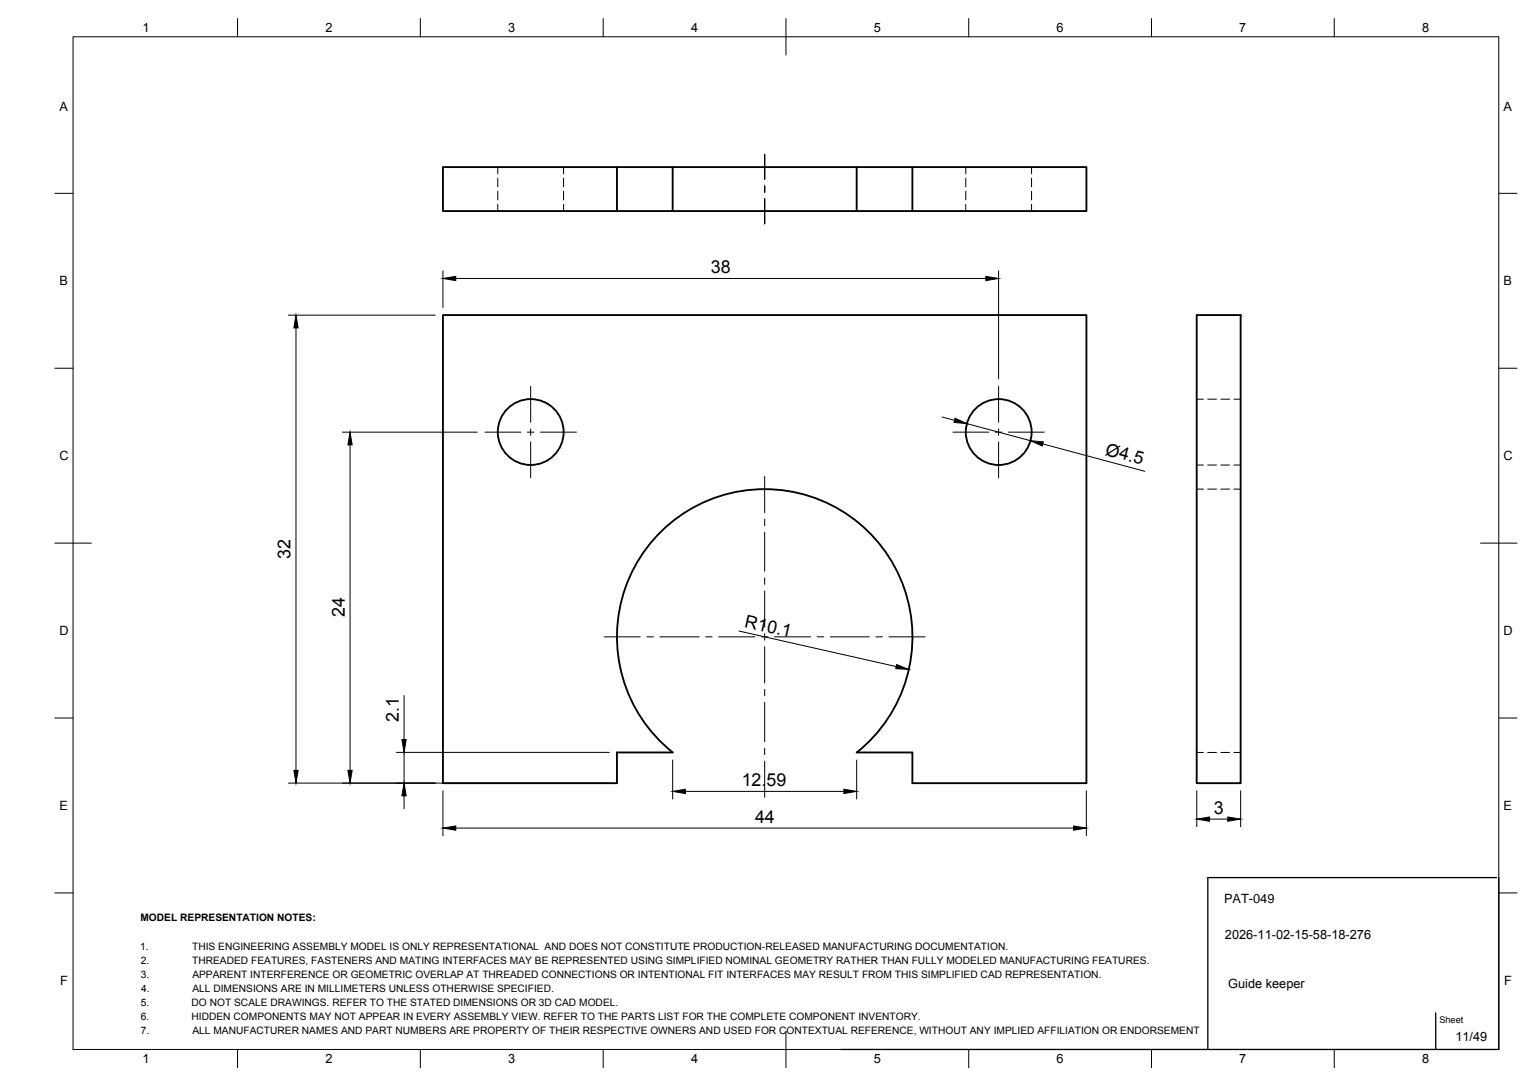
ISO-10303-21;
HEADER;
/* Generated by software containing ST-Developer
 * from STEP Tools, Inc. (www.steptools.com) 
 */

FILE_DESCRIPTION(
/* description */ ('Hand drill press frame (manual)'),
/* implementation_level */ '2;1');

FILE_NAME(
/* name */ 'Guide keeper.step',
/* time_stamp */ '2026-10-28T03:25:28-07:00',
/* author */ (''),
/* organization */ (''),
/* preprocessor_version */ 'ST-DEVELOPER v20.2',
/* originating_system */ 'Autodesk Translation Framework v15.17.0.0',
/* authorisation */ '');

FILE_SCHEMA (('AUTOMOTIVE_DESIGN { 1 0 10303 214 3 1 1 }'));
ENDSEC;

DATA;
#10=MECHANICAL_DESIGN_GEOMETRIC_PRESENTATION_REPRESENTATION('',(#625),#33299);
#535=SHAPE_REPRESENTATION_RELATIONSHIP('SRR','None',#33494,#580);
#580=ADVANCED_BREP_SHAPE_REPRESENTATION('',(#677),#33256);
#625=STYLED_ITEM('',(#33807),#677);
#677=MANIFOLD_SOLID_BREP('Body1',#12643);
#749=FACE_BOUND('',#2154,.T.);
#750=FACE_BOUND('',#2155,.T.);
#751=FACE_BOUND('',#2161,.T.);
#752=FACE_BOUND('',#2162,.T.);
#945=PLANE('',#13357);
#946=PLANE('',#13358);
#947=PLANE('',#13359);
#948=PLANE('',#13360);
#949=PLANE('',#13361);
#950=PLANE('',#13362);
#951=PLANE('',#13363);
#952=PLANE('',#13367);
#953=PLANE('',#13368);
#954=PLANE('',#13369);
#955=PLANE('',#13370);
#1427=FACE_OUTER_BOUND('',#2145,.T.);
#1428=FACE_OUTER_BOUND('',#2146,.T.);
#1429=FACE_OUTER_BOUND('',#2147,.T.);
#1430=FACE_OUTER_BOUND('',#2148,.T.);
#1431=FACE_OUTER_BOUND('',#2149,.T.);
#1432=FACE_OUTER_BOUND('',#2150,.T.);
#1433=FACE_OUTER_BOUND('',#2151,.T.);
#1434=FACE_OUTER_BOUND('',#2152,.T.);
#1435=FACE_OUTER_BOUND('',#2153,.T.);
#1436=FACE_OUTER_BOUND('',#2156,.T.);
#1437=FACE_OUTER_BOUND('',#2157,.T.);
#1438=FACE_OUTER_BOUND('',#2158,.T.);
#1439=FACE_OUTER_BOUND('',#2159,.T.);
#1440=FACE_OUTER_BOUND('',#2160,.T.);
#2145=EDGE_LOOP('',(#8835,#8836,#8837,#8838));
#2146=EDGE_LOOP('',(#8839,#8840,#8841,#8842));
#2147=EDGE_LOOP('',(#8843,#8844,#8845,#8846));
#2148=EDGE_LOOP('',(#8847,#8848,#8849,#8850));
#2149=EDGE_LOOP('',(#8851,#8852,#8853,#8854));
#2150=EDGE_LOOP('',(#8855,#8856,#8857,#8858));
#2151=EDGE_LOOP('',(#8859,#8860,#8861,#8862));
#2152=EDGE_LOOP('',(#8863,#8864,#8865,#8866));
#2153=EDGE_LOOP('',(#8867,#8868,#8869,#8870,#8871,#8872,#8873,#8874,#8875,
#8876));
#2154=EDGE_LOOP('',(#8877));
#2155=EDGE_LOOP('',(#8878));
#2156=EDGE_LOOP('',(#8879,#8880,#8881,#8882));
#2157=EDGE_LOOP('',(#8883,#8884,#8885,#8886));
#2158=EDGE_LOOP('',(#8887,#8888,#8889,#8890));
#2159=EDGE_LOOP('',(#8891,#8892,#8893,#8894));
#2160=EDGE_LOOP('',(#8895,#8896,#8897,#8898,#8899,#8900,#8901,#8902,#8903,
#8904));
#2161=EDGE_LOOP('',(#8905));
#2162=EDGE_LOOP('',(#8906));
#3015=LINE('',#18458,#4180);
#3016=LINE('',#18464,#4181);
#3017=LINE('',#18469,#4182);
#3018=LINE('',#18471,#4183);
#3019=LINE('',#18473,#4184);
#3020=LINE('',#18474,#4185);
#3021=LINE('',#18478,#4186);
#3022=LINE('',#18480,#4187);
#3023=LINE('',#18482,#4188);
#3024=LINE('',#18483,#4189);
#3025=LINE('',#18486,#4190);
#3026=LINE('',#18488,#4191);
#3027=LINE('',#18489,#4192);
#3028=LINE('',#18492,#4193);
#3029=LINE('',#18494,#4194);
#3030=LINE('',#18495,#4195);
#3031=LINE('',#18498,#4196);
#3032=LINE('',#18500,#4197);
#3033=LINE('',#18501,#4198);
#3034=LINE('',#18504,#4199);
#3035=LINE('',#18506,#4200);
#3036=LINE('',#18507,#4201);
#3037=LINE('',#18511,#4202);
#3038=LINE('',#18513,#4203);
#3039=LINE('',#18514,#4204);
#3040=LINE('',#18519,#4205);
#3041=LINE('',#18520,#4206);
#3042=LINE('',#18523,#4207);
#3043=LINE('',#18524,#4208);
#3044=LINE('',#18526,#4209);
#4180=VECTOR('',#14828,0.225);
#4181=VECTOR('',#14835,0.225);
#4182=VECTOR('',#14840,1.);
#4183=VECTOR('',#14841,1.);
#4184=VECTOR('',#14842,1.);
#4185=VECTOR('',#14843,1.);
#4186=VECTOR('',#14846,1.);
#4187=VECTOR('',#14847,1.);
#4188=VECTOR('',#14848,1.);
#4189=VECTOR('',#14849,1.);
#4190=VECTOR('',#14852,1.);
#4191=VECTOR('',#14853,1.);
#4192=VECTOR('',#14854,1.);
#4193=VECTOR('',#14857,1.);
#4194=VECTOR('',#14858,1.);
#4195=VECTOR('',#14859,1.);
#4196=VECTOR('',#14862,1.);
#4197=VECTOR('',#14863,1.);
#4198=VECTOR('',#14864,1.);
#4199=VECTOR('',#14867,1.);
#4200=VECTOR('',#14868,1.);
#4201=VECTOR('',#14869,1.);
#4202=VECTOR('',#14874,1.);
#4203=VECTOR('',#14875,1.);
#4204=VECTOR('',#14876,1.);
#4205=VECTOR('',#14883,1.);
#4206=VECTOR('',#14884,1.);
#4207=VECTOR('',#14887,1.);
#4208=VECTOR('',#14888,1.);
#4209=VECTOR('',#14891,1.);
#5280=CIRCLE('',#13352,0.225);
#5281=CIRCLE('',#13353,0.225);
#5282=CIRCLE('',#13355,0.225);
#5283=CIRCLE('',#13356,0.225);
#5284=CIRCLE('',#13364,1.01);
#5285=CIRCLE('',#13366,1.01);
#5751=VERTEX_POINT('',#18455);
#5752=VERTEX_POINT('',#18457);
#5753=VERTEX_POINT('',#18461);
#5754=VERTEX_POINT('',#18463);
#5755=VERTEX_POINT('',#18467);
#5756=VERTEX_POINT('',#18468);
#5757=VERTEX_POINT('',#18470);
#5758=VERTEX_POINT('',#18472);
#5759=VERTEX_POINT('',#18476);
#5760=VERTEX_POINT('',#18477);
#5761=VERTEX_POINT('',#18479);
#5762=VERTEX_POINT('',#18481);
#5763=VERTEX_POINT('',#18485);
#5764=VERTEX_POINT('',#18487);
#5765=VERTEX_POINT('',#18491);
#5766=VERTEX_POINT('',#18493);
#5767=VERTEX_POINT('',#18497);
#5768=VERTEX_POINT('',#18499);
#5769=VERTEX_POINT('',#18503);
#5770=VERTEX_POINT('',#18505);
#5771=VERTEX_POINT('',#18510);
#5772=VERTEX_POINT('',#18512);
#5773=VERTEX_POINT('',#18518);
#5774=VERTEX_POINT('',#18522);
#6946=EDGE_CURVE('',#5751,#5751,#5280,.T.);
#6947=EDGE_CURVE('',#5751,#5752,#3015,.T.);
#6948=EDGE_CURVE('',#5752,#5752,#5281,.T.);
#6949=EDGE_CURVE('',#5753,#5753,#5282,.T.);
#6950=EDGE_CURVE('',#5753,#5754,#3016,.T.);
#6951=EDGE_CURVE('',#5754,#5754,#5283,.T.);
#6952=EDGE_CURVE('',#5755,#5756,#3017,.T.);
#6953=EDGE_CURVE('',#5755,#5757,#3018,.T.);
#6954=EDGE_CURVE('',#5758,#5757,#3019,.T.);
#6955=EDGE_CURVE('',#5756,#5758,#3020,.T.);
#6956=EDGE_CURVE('',#5759,#5760,#3021,.T.);
#6957=EDGE_CURVE('',#5761,#5759,#3022,.T.);
#6958=EDGE_CURVE('',#5762,#5761,#3023,.T.);
#6959=EDGE_CURVE('',#5760,#5762,#3024,.T.);
#6960=EDGE_CURVE('',#5763,#5759,#3025,.T.);
#6961=EDGE_CURVE('',#5764,#5763,#3026,.T.);
#6962=EDGE_CURVE('',#5761,#5764,#3027,.T.);
#6963=EDGE_CURVE('',#5765,#5755,#3028,.T.);
#6964=EDGE_CURVE('',#5766,#5765,#3029,.T.);
#6965=EDGE_CURVE('',#5757,#5766,#3030,.T.);
#6966=EDGE_CURVE('',#5767,#5758,#3031,.T.);
#6967=EDGE_CURVE('',#5768,#5767,#3032,.T.);
#6968=EDGE_CURVE('',#5768,#5756,#3033,.T.);
#6969=EDGE_CURVE('',#5762,#5769,#3034,.T.);
#6970=EDGE_CURVE('',#5769,#5770,#3035,.T.);
#6971=EDGE_CURVE('',#5760,#5770,#3036,.T.);
#6972=EDGE_CURVE('',#5766,#5763,#5284,.T.);
#6973=EDGE_CURVE('',#5770,#5771,#3037,.T.);
#6974=EDGE_CURVE('',#5771,#5772,#3038,.T.);
#6975=EDGE_CURVE('',#5772,#5767,#3039,.T.);
#6976=EDGE_CURVE('',#5764,#5765,#5285,.T.);
#6977=EDGE_CURVE('',#5773,#5768,#3040,.T.);
#6978=EDGE_CURVE('',#5773,#5772,#3041,.T.);
#6979=EDGE_CURVE('',#5774,#5773,#3042,.T.);
#6980=EDGE_CURVE('',#5774,#5771,#3043,.T.);
#6981=EDGE_CURVE('',#5769,#5774,#3044,.T.);
#8835=ORIENTED_EDGE('',*,*,#6946,.F.);
#8836=ORIENTED_EDGE('',*,*,#6947,.T.);
#8837=ORIENTED_EDGE('',*,*,#6948,.F.);
#8838=ORIENTED_EDGE('',*,*,#6947,.F.);
#8839=ORIENTED_EDGE('',*,*,#6949,.F.);
#8840=ORIENTED_EDGE('',*,*,#6950,.T.);
#8841=ORIENTED_EDGE('',*,*,#6951,.F.);
#8842=ORIENTED_EDGE('',*,*,#6950,.F.);
#8843=ORIENTED_EDGE('',*,*,#6952,.F.);
#8844=ORIENTED_EDGE('',*,*,#6953,.T.);
#8845=ORIENTED_EDGE('',*,*,#6954,.F.);
#8846=ORIENTED_EDGE('',*,*,#6955,.F.);
#8847=ORIENTED_EDGE('',*,*,#6956,.F.);
#8848=ORIENTED_EDGE('',*,*,#6957,.F.);
#8849=ORIENTED_EDGE('',*,*,#6958,.F.);
#8850=ORIENTED_EDGE('',*,*,#6959,.F.);
#8851=ORIENTED_EDGE('',*,*,#6960,.F.);
#8852=ORIENTED_EDGE('',*,*,#6961,.F.);
#8853=ORIENTED_EDGE('',*,*,#6962,.F.);
#8854=ORIENTED_EDGE('',*,*,#6957,.T.);
#8855=ORIENTED_EDGE('',*,*,#6963,.F.);
#8856=ORIENTED_EDGE('',*,*,#6964,.F.);
#8857=ORIENTED_EDGE('',*,*,#6965,.F.);
#8858=ORIENTED_EDGE('',*,*,#6953,.F.);
#8859=ORIENTED_EDGE('',*,*,#6955,.T.);
#8860=ORIENTED_EDGE('',*,*,#6966,.F.);
#8861=ORIENTED_EDGE('',*,*,#6967,.F.);
#8862=ORIENTED_EDGE('',*,*,#6968,.T.);
#8863=ORIENTED_EDGE('',*,*,#6959,.T.);
#8864=ORIENTED_EDGE('',*,*,#6969,.T.);
#8865=ORIENTED_EDGE('',*,*,#6970,.T.);
#8866=ORIENTED_EDGE('',*,*,#6971,.F.);
#8867=ORIENTED_EDGE('',*,*,#6954,.T.);
#8868=ORIENTED_EDGE('',*,*,#6965,.T.);
#8869=ORIENTED_EDGE('',*,*,#6972,.T.);
#8870=ORIENTED_EDGE('',*,*,#6960,.T.);
#8871=ORIENTED_EDGE('',*,*,#6956,.T.);
#8872=ORIENTED_EDGE('',*,*,#6971,.T.);
#8873=ORIENTED_EDGE('',*,*,#6973,.T.);
#8874=ORIENTED_EDGE('',*,*,#6974,.T.);
#8875=ORIENTED_EDGE('',*,*,#6975,.T.);
#8876=ORIENTED_EDGE('',*,*,#6966,.T.);
#8877=ORIENTED_EDGE('',*,*,#6948,.T.);
#8878=ORIENTED_EDGE('',*,*,#6951,.T.);
#8879=ORIENTED_EDGE('',*,*,#6964,.T.);
#8880=ORIENTED_EDGE('',*,*,#6976,.F.);
#8881=ORIENTED_EDGE('',*,*,#6961,.T.);
#8882=ORIENTED_EDGE('',*,*,#6972,.F.);
#8883=ORIENTED_EDGE('',*,*,#6977,.T.);
#8884=ORIENTED_EDGE('',*,*,#6967,.T.);
#8885=ORIENTED_EDGE('',*,*,#6975,.F.);
#8886=ORIENTED_EDGE('',*,*,#6978,.F.);
#8887=ORIENTED_EDGE('',*,*,#6979,.T.);
#8888=ORIENTED_EDGE('',*,*,#6978,.T.);
#8889=ORIENTED_EDGE('',*,*,#6974,.F.);
#8890=ORIENTED_EDGE('',*,*,#6980,.F.);
#8891=ORIENTED_EDGE('',*,*,#6981,.T.);
#8892=ORIENTED_EDGE('',*,*,#6980,.T.);
#8893=ORIENTED_EDGE('',*,*,#6973,.F.);
#8894=ORIENTED_EDGE('',*,*,#6970,.F.);
#8895=ORIENTED_EDGE('',*,*,#6952,.T.);
#8896=ORIENTED_EDGE('',*,*,#6968,.F.);
#8897=ORIENTED_EDGE('',*,*,#6977,.F.);
#8898=ORIENTED_EDGE('',*,*,#6979,.F.);
#8899=ORIENTED_EDGE('',*,*,#6981,.F.);
#8900=ORIENTED_EDGE('',*,*,#6969,.F.);
#8901=ORIENTED_EDGE('',*,*,#6958,.T.);
#8902=ORIENTED_EDGE('',*,*,#6962,.T.);
#8903=ORIENTED_EDGE('',*,*,#6976,.T.);
#8904=ORIENTED_EDGE('',*,*,#6963,.T.);
#8905=ORIENTED_EDGE('',*,*,#6946,.T.);
#8906=ORIENTED_EDGE('',*,*,#6949,.T.);
#11815=CYLINDRICAL_SURFACE('',#13351,0.225);
#11816=CYLINDRICAL_SURFACE('',#13354,0.225);
#11817=CYLINDRICAL_SURFACE('',#13365,1.01);
#12036=ADVANCED_FACE('',(#1427),#11815,.F.);
#12037=ADVANCED_FACE('',(#1428),#11816,.F.);
#12038=ADVANCED_FACE('',(#1429),#945,.F.);
#12039=ADVANCED_FACE('',(#1430),#946,.F.);
#12040=ADVANCED_FACE('',(#1431),#947,.F.);
#12041=ADVANCED_FACE('',(#1432),#948,.F.);
#12042=ADVANCED_FACE('',(#1433),#949,.T.);
#12043=ADVANCED_FACE('',(#1434),#950,.T.);
#12044=ADVANCED_FACE('',(#1435,#749,#750),#951,.T.);
#12045=ADVANCED_FACE('',(#1436),#11817,.F.);
#12046=ADVANCED_FACE('',(#1437),#952,.T.);
#12047=ADVANCED_FACE('',(#1438),#953,.T.);
#12048=ADVANCED_FACE('',(#1439),#954,.T.);
#12049=ADVANCED_FACE('',(#1440,#751,#752),#955,.F.);
#12643=CLOSED_SHELL('',(#12036,#12037,#12038,#12039,#12040,#12041,#12042,
#12043,#12044,#12045,#12046,#12047,#12048,#12049));
#13350=AXIS2_PLACEMENT_3D('',#18453,#14822,#14823);
#13351=AXIS2_PLACEMENT_3D('',#18454,#14824,#14825);
#13352=AXIS2_PLACEMENT_3D('',#18456,#14826,#14827);
#13353=AXIS2_PLACEMENT_3D('',#18459,#14829,#14830);
#13354=AXIS2_PLACEMENT_3D('',#18460,#14831,#14832);
#13355=AXIS2_PLACEMENT_3D('',#18462,#14833,#14834);
#13356=AXIS2_PLACEMENT_3D('',#18465,#14836,#14837);
#13357=AXIS2_PLACEMENT_3D('',#18466,#14838,#14839);
#13358=AXIS2_PLACEMENT_3D('',#18475,#14844,#14845);
#13359=AXIS2_PLACEMENT_3D('',#18484,#14850,#14851);
#13360=AXIS2_PLACEMENT_3D('',#18490,#14855,#14856);
#13361=AXIS2_PLACEMENT_3D('',#18496,#14860,#14861);
#13362=AXIS2_PLACEMENT_3D('',#18502,#14865,#14866);
#13363=AXIS2_PLACEMENT_3D('',#18508,#14870,#14871);
#13364=AXIS2_PLACEMENT_3D('',#18509,#14872,#14873);
#13365=AXIS2_PLACEMENT_3D('',#18515,#14877,#14878);
#13366=AXIS2_PLACEMENT_3D('',#18516,#14879,#14880);
#13367=AXIS2_PLACEMENT_3D('',#18517,#14881,#14882);
#13368=AXIS2_PLACEMENT_3D('',#18521,#14885,#14886);
#13369=AXIS2_PLACEMENT_3D('',#18525,#14889,#14890);
#13370=AXIS2_PLACEMENT_3D('',#18527,#14892,#14893);
#14822=DIRECTION('axis',(0.,0.,1.));
#14823=DIRECTION('refdir',(1.,0.,0.));
#14824=DIRECTION('center_axis',(0.,0.,1.));
#14825=DIRECTION('ref_axis',(1.,0.,0.));
#14826=DIRECTION('center_axis',(0.,0.,1.));
#14827=DIRECTION('ref_axis',(1.,0.,0.));
#14828=DIRECTION('',(0.,0.,1.));
#14829=DIRECTION('center_axis',(0.,0.,-1.));
#14830=DIRECTION('ref_axis',(1.,0.,0.));
#14831=DIRECTION('center_axis',(0.,0.,1.));
#14832=DIRECTION('ref_axis',(1.,0.,0.));
#14833=DIRECTION('center_axis',(0.,0.,1.));
#14834=DIRECTION('ref_axis',(1.,0.,0.));
#14835=DIRECTION('',(0.,0.,1.));
#14836=DIRECTION('center_axis',(0.,0.,-1.));
#14837=DIRECTION('ref_axis',(1.,0.,0.));
#14838=DIRECTION('center_axis',(0.,1.,0.));
#14839=DIRECTION('ref_axis',(-1.,0.,0.));
#14840=DIRECTION('',(-1.,0.,0.));
#14841=DIRECTION('',(0.,0.,1.));
#14842=DIRECTION('',(1.,0.,0.));
#14843=DIRECTION('',(0.,0.,1.));
#14844=DIRECTION('center_axis',(0.,-1.,0.));
#14845=DIRECTION('ref_axis',(1.,0.,0.));
#14846=DIRECTION('',(-1.,0.,0.));
#14847=DIRECTION('',(0.,0.,1.));
#14848=DIRECTION('',(1.,0.,0.));
#14849=DIRECTION('',(0.,0.,-1.));
#14850=DIRECTION('center_axis',(1.,0.,0.));
#14851=DIRECTION('ref_axis',(0.,1.,0.));
#14852=DIRECTION('',(0.,-1.,0.));
#14853=DIRECTION('',(0.,0.,1.));
#14854=DIRECTION('',(0.,1.,0.));
#14855=DIRECTION('center_axis',(1.,0.,0.));
#14856=DIRECTION('ref_axis',(0.,1.,0.));
#14857=DIRECTION('',(0.,1.,0.));
#14858=DIRECTION('',(0.,0.,-1.));
#14859=DIRECTION('',(0.,-1.,0.));
#14860=DIRECTION('center_axis',(-1.,0.,0.));
#14861=DIRECTION('ref_axis',(0.,-1.,0.));
#14862=DIRECTION('',(0.,-1.,0.));
#14863=DIRECTION('',(0.,0.,1.));
#14864=DIRECTION('',(0.,-1.,0.));
#14865=DIRECTION('center_axis',(-1.,0.,0.));
#14866=DIRECTION('ref_axis',(0.,-1.,0.));
#14867=DIRECTION('',(0.,-1.,0.));
#14868=DIRECTION('',(0.,0.,1.));
#14869=DIRECTION('',(0.,-1.,0.));
#14870=DIRECTION('center_axis',(0.,0.,1.));
#14871=DIRECTION('ref_axis',(1.,0.,0.));
#14872=DIRECTION('center_axis',(0.,0.,-1.));
#14873=DIRECTION('ref_axis',(1.,0.,0.));
#14874=DIRECTION('',(1.,0.,0.));
#14875=DIRECTION('',(0.,1.,0.));
#14876=DIRECTION('',(-1.,0.,0.));
#14877=DIRECTION('center_axis',(0.,0.,1.));
#14878=DIRECTION('ref_axis',(1.,0.,0.));
#14879=DIRECTION('center_axis',(0.,0.,1.));
#14880=DIRECTION('ref_axis',(1.,0.,0.));
#14881=DIRECTION('center_axis',(0.,1.,0.));
#14882=DIRECTION('ref_axis',(-1.,0.,0.));
#14883=DIRECTION('',(-1.,0.,0.));
#14884=DIRECTION('',(0.,0.,1.));
#14885=DIRECTION('center_axis',(1.,0.,0.));
#14886=DIRECTION('ref_axis',(0.,1.,0.));
#14887=DIRECTION('',(0.,1.,0.));
#14888=DIRECTION('',(0.,0.,1.));
#14889=DIRECTION('center_axis',(0.,-1.,0.));
#14890=DIRECTION('ref_axis',(1.,0.,0.));
#14891=DIRECTION('',(1.,0.,0.));
#14892=DIRECTION('center_axis',(0.,0.,1.));
#14893=DIRECTION('ref_axis',(1.,0.,0.));
#18453=CARTESIAN_POINT('',(0.,0.,0.));
#18454=CARTESIAN_POINT('Origin',(2.4,-1.6,15.2));
#18455=CARTESIAN_POINT('',(2.175,-1.6,15.3));
#18456=CARTESIAN_POINT('Origin',(2.4,-1.6,15.3));
#18457=CARTESIAN_POINT('',(2.175,-1.6,15.6));
#18458=CARTESIAN_POINT('',(2.175,-1.6,15.2));
#18459=CARTESIAN_POINT('Origin',(2.4,-1.6,15.6));
#18460=CARTESIAN_POINT('Origin',(2.4,1.6,15.2));
#18461=CARTESIAN_POINT('',(2.175,1.6,15.3));
#18462=CARTESIAN_POINT('Origin',(2.4,1.6,15.3));
#18463=CARTESIAN_POINT('',(2.175,1.6,15.6));
#18464=CARTESIAN_POINT('',(2.175,1.6,15.2));
#18465=CARTESIAN_POINT('Origin',(2.4,1.6,15.6));
#18466=CARTESIAN_POINT('Origin',(0.21,1.01,15.2));
#18467=CARTESIAN_POINT('',(0.21,1.01,15.3));
#18468=CARTESIAN_POINT('',(0.,1.01,15.3));
#18469=CARTESIAN_POINT('',(0.905,1.01,15.3));
#18470=CARTESIAN_POINT('',(0.21,1.01,15.6));
#18471=CARTESIAN_POINT('',(0.21,1.01,15.2));
#18472=CARTESIAN_POINT('',(0.,1.01,15.6));
#18473=CARTESIAN_POINT('',(0.905,1.01,15.6));
#18474=CARTESIAN_POINT('',(0.,1.01,15.25));
#18475=CARTESIAN_POINT('Origin',(-0.1,-1.01,15.2));
#18476=CARTESIAN_POINT('',(0.21,-1.01,15.6));
#18477=CARTESIAN_POINT('',(0.,-1.01,15.6));
#18478=CARTESIAN_POINT('',(0.75,-1.01,15.6));
#18479=CARTESIAN_POINT('',(0.21,-1.01,15.3));
#18480=CARTESIAN_POINT('',(0.21,-1.01,15.2));
#18481=CARTESIAN_POINT('',(0.,-1.01,15.3));
#18482=CARTESIAN_POINT('',(0.75,-1.01,15.3));
#18483=CARTESIAN_POINT('',(0.,-1.01,15.25));
#18484=CARTESIAN_POINT('Origin',(0.21,-1.01,15.2));
#18485=CARTESIAN_POINT('',(0.21,-0.629285308902091,15.6));
#18486=CARTESIAN_POINT('',(0.21,-0.505,15.6));
#18487=CARTESIAN_POINT('',(0.21,-0.629285308902091,15.3));
#18488=CARTESIAN_POINT('',(0.21,-0.629285308902091,15.2));
#18489=CARTESIAN_POINT('',(0.21,-0.505,15.3));
#18490=CARTESIAN_POINT('Origin',(0.21,-1.01,15.2));
#18491=CARTESIAN_POINT('',(0.21,0.629285308902091,15.3));
#18492=CARTESIAN_POINT('',(0.21,-0.505,15.3));
#18493=CARTESIAN_POINT('',(0.21,0.629285308902091,15.6));
#18494=CARTESIAN_POINT('',(0.21,0.629285308902091,15.2));
#18495=CARTESIAN_POINT('',(0.21,-0.505,15.6));
#18496=CARTESIAN_POINT('Origin',(0.,2.2,15.3));
#18497=CARTESIAN_POINT('',(0.,2.2,15.6));
#18498=CARTESIAN_POINT('',(0.,2.2,15.6));
#18499=CARTESIAN_POINT('',(0.,2.2,15.3));
#18500=CARTESIAN_POINT('',(0.,2.2,15.3));
#18501=CARTESIAN_POINT('',(0.,2.2,15.3));
#18502=CARTESIAN_POINT('Origin',(0.,2.2,15.3));
#18503=CARTESIAN_POINT('',(0.,-2.2,15.3));
#18504=CARTESIAN_POINT('',(0.,2.2,15.3));
#18505=CARTESIAN_POINT('',(0.,-2.2,15.6));
#18506=CARTESIAN_POINT('',(0.,-2.2,15.3));
#18507=CARTESIAN_POINT('',(0.,2.2,15.6));
#18508=CARTESIAN_POINT('Origin',(1.6,0.,15.6));
#18509=CARTESIAN_POINT('Origin',(1.,0.,15.6));
#18510=CARTESIAN_POINT('',(3.2,-2.2,15.6));
#18511=CARTESIAN_POINT('',(0.,-2.2,15.6));
#18512=CARTESIAN_POINT('',(3.2,2.2,15.6));
#18513=CARTESIAN_POINT('',(3.2,-2.2,15.6));
#18514=CARTESIAN_POINT('',(3.2,2.2,15.6));
#18515=CARTESIAN_POINT('Origin',(1.,0.,15.2));
#18516=CARTESIAN_POINT('Origin',(1.,0.,15.3));
#18517=CARTESIAN_POINT('Origin',(3.2,2.2,15.3));
#18518=CARTESIAN_POINT('',(3.2,2.2,15.3));
#18519=CARTESIAN_POINT('',(3.2,2.2,15.3));
#18520=CARTESIAN_POINT('',(3.2,2.2,15.3));
#18521=CARTESIAN_POINT('Origin',(3.2,-2.2,15.3));
#18522=CARTESIAN_POINT('',(3.2,-2.2,15.3));
#18523=CARTESIAN_POINT('',(3.2,-2.2,15.3));
#18524=CARTESIAN_POINT('',(3.2,-2.2,15.3));
#18525=CARTESIAN_POINT('Origin',(0.,-2.2,15.3));
#18526=CARTESIAN_POINT('',(0.,-2.2,15.3));
#18527=CARTESIAN_POINT('Origin',(1.6,0.,15.3));
#33204=UNCERTAINTY_MEASURE_WITH_UNIT(LENGTH_MEASURE(0.001),#33300,
'DISTANCE_ACCURACY_VALUE',
'Maximum model space distance between geometric entities at asserted c
onnectivities');
#33247=UNCERTAINTY_MEASURE_WITH_UNIT(LENGTH_MEASURE(0.001),#33300,
'DISTANCE_ACCURACY_VALUE',
'Maximum model space distance between geometric entities at asserted c
onnectivities');
#33256=(
GEOMETRIC_REPRESENTATION_CONTEXT(3)
GLOBAL_UNCERTAINTY_ASSIGNED_CONTEXT((#33204))
GLOBAL_UNIT_ASSIGNED_CONTEXT((#33300,#33302,#33303))
REPRESENTATION_CONTEXT('','3D')
);
#33299=(
GEOMETRIC_REPRESENTATION_CONTEXT(3)
GLOBAL_UNCERTAINTY_ASSIGNED_CONTEXT((#33247))
GLOBAL_UNIT_ASSIGNED_CONTEXT((#33300,#33302,#33303))
REPRESENTATION_CONTEXT('','3D')
);
#33300=(
LENGTH_UNIT()
NAMED_UNIT(*)
SI_UNIT(.CENTI.,.METRE.)
);
#33302=(
NAMED_UNIT(*)
PLANE_ANGLE_UNIT()
SI_UNIT($,.RADIAN.)
);
#33303=(
NAMED_UNIT(*)
SI_UNIT($,.STERADIAN.)
SOLID_ANGLE_UNIT()
);
#33312=SHAPE_DEFINITION_REPRESENTATION(#33363,#33494);
#33363=PRODUCT_DEFINITION_SHAPE('',$,#33546);
#33494=SHAPE_REPRESENTATION('',(#13350),#33256);
#33537=PRODUCT_DEFINITION_CONTEXT('part definition',#33692,'design');
#33546=PRODUCT_DEFINITION('Guide keeper','Guide keeper',#33597,#33537);
#33597=PRODUCT_DEFINITION_FORMATION('',$,#33702);
#33692=APPLICATION_CONTEXT(
'Core Data for Automotive Mechanical Design Process');
#33693=PRODUCT_CONTEXT('part definition',#33692,'mechanical');
#33702=PRODUCT('Guide keeper','Guide keeper','Guide keeper',(#33693));
#33801=COLOUR_RGB('Sky Blue',0.24,0.69,0.87);
#33802=FILL_AREA_STYLE_COLOUR('',#33801);
#33803=FILL_AREA_STYLE('',(#33802));
#33804=SURFACE_STYLE_FILL_AREA(#33803);
#33805=SURFACE_SIDE_STYLE('',(#33804));
#33806=SURFACE_STYLE_USAGE(.BOTH.,#33805);
#33807=PRESENTATION_STYLE_ASSIGNMENT((#33806));
ENDSEC;
END-ISO-10303-21;
